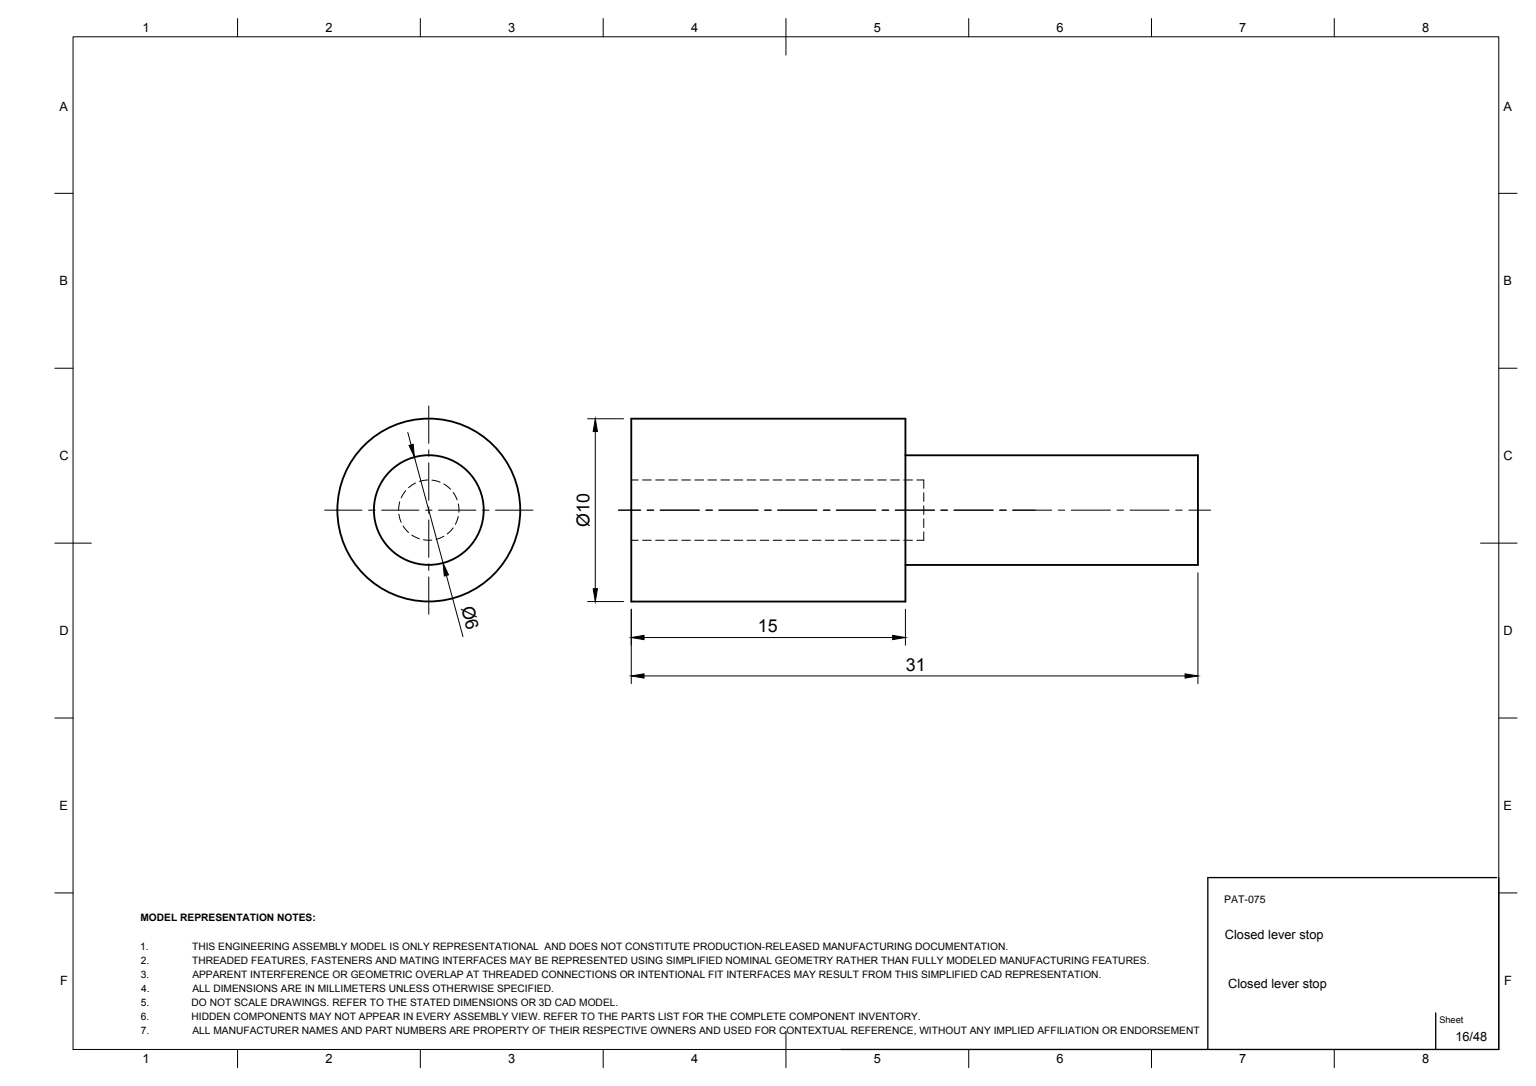
ISO-10303-21;
HEADER;
/* Generated by software containing ST-Developer
 * from STEP Tools, Inc. (www.steptools.com) 
 */

FILE_DESCRIPTION(
/* description */ ('Over-Centre Plunger Toggle Clamp on Slotted Fixture Frame'),
/* implementation_level */ '2;1');

FILE_NAME(
/* name */ 
'Closed lever stop.step',
/* time_stamp */ '2026-10-28T03:23:24-07:00',
/* author */ (''),
/* organization */ (''),
/* preprocessor_version */ 'ST-DEVELOPER v20.2',
/* originating_system */ 'Autodesk Translation Framework v15.17.0.0',
/* authorisation */ '');

FILE_SCHEMA (('AUTOMOTIVE_DESIGN { 1 0 10303 214 3 1 1 }'));
ENDSEC;

DATA;
#10=MECHANICAL_DESIGN_GEOMETRIC_PRESENTATION_REPRESENTATION('',(#524),#15212);
#440=SHAPE_REPRESENTATION_RELATIONSHIP('SRR','None',#15414,#482);
#482=ADVANCED_BREP_SHAPE_REPRESENTATION('',(#575),#15176);
#524=STYLED_ITEM('',(#15712),#575);
#575=MANIFOLD_SOLID_BREP('Body1',#8256);
#712=FACE_BOUND('',#1819,.T.);
#713=FACE_BOUND('',#1822,.T.);
#862=PLANE('',#9048);
#863=PLANE('',#9049);
#864=PLANE('',#9054);
#865=PLANE('',#9057);
#1229=FACE_OUTER_BOUND('',#1816,.T.);
#1230=FACE_OUTER_BOUND('',#1817,.T.);
#1231=FACE_OUTER_BOUND('',#1818,.T.);
#1232=FACE_OUTER_BOUND('',#1820,.T.);
#1233=FACE_OUTER_BOUND('',#1821,.T.);
#1234=FACE_OUTER_BOUND('',#1823,.T.);
#1235=FACE_OUTER_BOUND('',#1824,.T.);
#1816=EDGE_LOOP('',(#6187,#6188,#6189,#6190));
#1817=EDGE_LOOP('',(#6191));
#1818=EDGE_LOOP('',(#6192));
#1819=EDGE_LOOP('',(#6193));
#1820=EDGE_LOOP('',(#6194,#6195,#6196,#6197));
#1821=EDGE_LOOP('',(#6198));
#1822=EDGE_LOOP('',(#6199));
#1823=EDGE_LOOP('',(#6200,#6201,#6202,#6203));
#1824=EDGE_LOOP('',(#6204));
#2414=LINE('',#13041,#3044);
#2415=LINE('',#13052,#3045);
#2416=LINE('',#13056,#3046);
#3044=VECTOR('',#10505,0.165);
#3045=VECTOR('',#10520,0.5);
#3046=VECTOR('',#10525,0.3);
#3617=CIRCLE('',#9046,0.165);
#3618=CIRCLE('',#9047,0.165);
#3619=CIRCLE('',#9050,0.5);
#3620=CIRCLE('',#9051,0.3);
#3621=CIRCLE('',#9053,0.5);
#3622=CIRCLE('',#9056,0.3);
#4065=VERTEX_POINT('',#13038);
#4066=VERTEX_POINT('',#13040);
#4067=VERTEX_POINT('',#13045);
#4068=VERTEX_POINT('',#13047);
#4069=VERTEX_POINT('',#13050);
#4070=VERTEX_POINT('',#13055);
#4854=EDGE_CURVE('',#4065,#4065,#3617,.T.);
#4855=EDGE_CURVE('',#4065,#4066,#2414,.T.);
#4856=EDGE_CURVE('',#4066,#4066,#3618,.T.);
#4857=EDGE_CURVE('',#4067,#4067,#3619,.T.);
#4858=EDGE_CURVE('',#4068,#4068,#3620,.T.);
#4859=EDGE_CURVE('',#4069,#4069,#3621,.T.);
#4860=EDGE_CURVE('',#4069,#4067,#2415,.T.);
#4861=EDGE_CURVE('',#4068,#4070,#2416,.T.);
#4862=EDGE_CURVE('',#4070,#4070,#3622,.T.);
#6187=ORIENTED_EDGE('',*,*,#4854,.F.);
#6188=ORIENTED_EDGE('',*,*,#4855,.T.);
#6189=ORIENTED_EDGE('',*,*,#4856,.F.);
#6190=ORIENTED_EDGE('',*,*,#4855,.F.);
#6191=ORIENTED_EDGE('',*,*,#4854,.T.);
#6192=ORIENTED_EDGE('',*,*,#4857,.F.);
#6193=ORIENTED_EDGE('',*,*,#4858,.T.);
#6194=ORIENTED_EDGE('',*,*,#4859,.F.);
#6195=ORIENTED_EDGE('',*,*,#4860,.T.);
#6196=ORIENTED_EDGE('',*,*,#4857,.T.);
#6197=ORIENTED_EDGE('',*,*,#4860,.F.);
#6198=ORIENTED_EDGE('',*,*,#4859,.T.);
#6199=ORIENTED_EDGE('',*,*,#4856,.T.);
#6200=ORIENTED_EDGE('',*,*,#4858,.F.);
#6201=ORIENTED_EDGE('',*,*,#4861,.T.);
#6202=ORIENTED_EDGE('',*,*,#4862,.T.);
#6203=ORIENTED_EDGE('',*,*,#4861,.F.);
#6204=ORIENTED_EDGE('',*,*,#4862,.F.);
#7680=CYLINDRICAL_SURFACE('',#9045,0.165);
#7681=CYLINDRICAL_SURFACE('',#9052,0.5);
#7682=CYLINDRICAL_SURFACE('',#9055,0.3);
#7901=ADVANCED_FACE('',(#1229),#7680,.F.);
#7902=ADVANCED_FACE('',(#1230),#862,.T.);
#7903=ADVANCED_FACE('',(#1231,#712),#863,.F.);
#7904=ADVANCED_FACE('',(#1232),#7681,.T.);
#7905=ADVANCED_FACE('',(#1233,#713),#864,.T.);
#7906=ADVANCED_FACE('',(#1234),#7682,.T.);
#7907=ADVANCED_FACE('',(#1235),#865,.F.);
#8256=CLOSED_SHELL('',(#7901,#7902,#7903,#7904,#7905,#7906,#7907));
#9044=AXIS2_PLACEMENT_3D('',#13036,#10499,#10500);
#9045=AXIS2_PLACEMENT_3D('',#13037,#10501,#10502);
#9046=AXIS2_PLACEMENT_3D('',#13039,#10503,#10504);
#9047=AXIS2_PLACEMENT_3D('',#13042,#10506,#10507);
#9048=AXIS2_PLACEMENT_3D('',#13043,#10508,#10509);
#9049=AXIS2_PLACEMENT_3D('',#13044,#10510,#10511);
#9050=AXIS2_PLACEMENT_3D('',#13046,#10512,#10513);
#9051=AXIS2_PLACEMENT_3D('',#13048,#10514,#10515);
#9052=AXIS2_PLACEMENT_3D('',#13049,#10516,#10517);
#9053=AXIS2_PLACEMENT_3D('',#13051,#10518,#10519);
#9054=AXIS2_PLACEMENT_3D('',#13053,#10521,#10522);
#9055=AXIS2_PLACEMENT_3D('',#13054,#10523,#10524);
#9056=AXIS2_PLACEMENT_3D('',#13057,#10526,#10527);
#9057=AXIS2_PLACEMENT_3D('',#13058,#10528,#10529);
#10499=DIRECTION('axis',(0.,0.,1.));
#10500=DIRECTION('refdir',(1.,0.,0.));
#10501=DIRECTION('center_axis',(0.,1.,0.));
#10502=DIRECTION('ref_axis',(1.,0.,0.));
#10503=DIRECTION('center_axis',(0.,1.,0.));
#10504=DIRECTION('ref_axis',(1.,0.,0.));
#10505=DIRECTION('',(0.,1.,0.));
#10506=DIRECTION('center_axis',(0.,-1.,0.));
#10507=DIRECTION('ref_axis',(1.,0.,0.));
#10508=DIRECTION('center_axis',(0.,1.,0.));
#10509=DIRECTION('ref_axis',(1.,0.,0.));
#10510=DIRECTION('center_axis',(0.,1.,0.));
#10511=DIRECTION('ref_axis',(1.,0.,0.));
#10512=DIRECTION('center_axis',(0.,1.,0.));
#10513=DIRECTION('ref_axis',(1.,0.,0.));
#10514=DIRECTION('center_axis',(0.,1.,0.));
#10515=DIRECTION('ref_axis',(1.,0.,0.));
#10516=DIRECTION('center_axis',(0.,1.,0.));
#10517=DIRECTION('ref_axis',(1.,0.,0.));
#10518=DIRECTION('center_axis',(0.,1.,0.));
#10519=DIRECTION('ref_axis',(1.,0.,0.));
#10520=DIRECTION('',(0.,-1.,0.));
#10521=DIRECTION('center_axis',(0.,1.,0.));
#10522=DIRECTION('ref_axis',(1.,0.,0.));
#10523=DIRECTION('center_axis',(0.,1.,0.));
#10524=DIRECTION('ref_axis',(1.,0.,0.));
#10525=DIRECTION('',(0.,-1.,0.));
#10526=DIRECTION('center_axis',(0.,1.,0.));
#10527=DIRECTION('ref_axis',(1.,0.,0.));
#10528=DIRECTION('center_axis',(0.,1.,0.));
#10529=DIRECTION('ref_axis',(1.,0.,0.));
#13036=CARTESIAN_POINT('',(0.,0.,0.));
#13037=CARTESIAN_POINT('Origin',(-5.25982293614231,-2.4,14.8604204653858));
#13038=CARTESIAN_POINT('',(-5.42482293614231,-2.4,14.8604204653858));
#13039=CARTESIAN_POINT('Origin',(-5.25982293614231,-2.4,14.8604204653858));
#13040=CARTESIAN_POINT('',(-5.42482293614231,-0.8,14.8604204653858));
#13041=CARTESIAN_POINT('',(-5.42482293614231,-2.4,14.8604204653858));
#13042=CARTESIAN_POINT('Origin',(-5.25982293614231,-0.8,14.8604204653858));
#13043=CARTESIAN_POINT('Origin',(-5.25982293614231,-2.4,14.8604204653858));
#13044=CARTESIAN_POINT('Origin',(-5.25982293614231,-2.3,14.8604204653858));
#13045=CARTESIAN_POINT('',(-5.75982293614231,-2.3,14.8604204653858));
#13046=CARTESIAN_POINT('Origin',(-5.25982293614231,-2.3,14.8604204653858));
#13047=CARTESIAN_POINT('',(-5.55982293614231,-2.3,14.8604204653858));
#13048=CARTESIAN_POINT('Origin',(-5.25982293614231,-2.3,14.8604204653858));
#13049=CARTESIAN_POINT('Origin',(-5.25982293614231,-2.3,14.8604204653858));
#13050=CARTESIAN_POINT('',(-5.75982293614231,-0.8,14.8604204653858));
#13051=CARTESIAN_POINT('Origin',(-5.25982293614231,-0.8,14.8604204653858));
#13052=CARTESIAN_POINT('',(-5.75982293614231,-2.3,14.8604204653858));
#13053=CARTESIAN_POINT('Origin',(-5.25982293614231,-0.8,14.8604204653858));
#13054=CARTESIAN_POINT('Origin',(-5.25982293614231,-3.9,14.8604204653858));
#13055=CARTESIAN_POINT('',(-5.55982293614231,-3.9,14.8604204653858));
#13056=CARTESIAN_POINT('',(-5.55982293614231,-3.9,14.8604204653858));
#13057=CARTESIAN_POINT('Origin',(-5.25982293614231,-3.9,14.8604204653858));
#13058=CARTESIAN_POINT('Origin',(-5.25982293614231,-3.9,14.8604204653858));
#15126=UNCERTAINTY_MEASURE_WITH_UNIT(LENGTH_MEASURE(0.001),#15213,
'DISTANCE_ACCURACY_VALUE',
'Maximum model space distance between geometric entities at asserted c
onnectivities');
#15162=UNCERTAINTY_MEASURE_WITH_UNIT(LENGTH_MEASURE(0.001),#15213,
'DISTANCE_ACCURACY_VALUE',
'Maximum model space distance between geometric entities at asserted c
onnectivities');
#15176=(
GEOMETRIC_REPRESENTATION_CONTEXT(3)
GLOBAL_UNCERTAINTY_ASSIGNED_CONTEXT((#15126))
GLOBAL_UNIT_ASSIGNED_CONTEXT((#15213,#15215,#15216))
REPRESENTATION_CONTEXT('','3D')
);
#15212=(
GEOMETRIC_REPRESENTATION_CONTEXT(3)
GLOBAL_UNCERTAINTY_ASSIGNED_CONTEXT((#15162))
GLOBAL_UNIT_ASSIGNED_CONTEXT((#15213,#15215,#15216))
REPRESENTATION_CONTEXT('','3D')
);
#15213=(
LENGTH_UNIT()
NAMED_UNIT(*)
SI_UNIT(.CENTI.,.METRE.)
);
#15215=(
NAMED_UNIT(*)
PLANE_ANGLE_UNIT()
SI_UNIT($,.RADIAN.)
);
#15216=(
NAMED_UNIT(*)
SI_UNIT($,.STERADIAN.)
SOLID_ANGLE_UNIT()
);
#15230=SHAPE_DEFINITION_REPRESENTATION(#15279,#15414);
#15279=PRODUCT_DEFINITION_SHAPE('',$,#15464);
#15414=SHAPE_REPRESENTATION('',(#9044),#15176);
#15450=PRODUCT_DEFINITION_CONTEXT('part definition',#15599,'design');
#15464=PRODUCT_DEFINITION('Closed lever stop','Closed lever stop',#15513,
#15450);
#15513=PRODUCT_DEFINITION_FORMATION('',$,#15614);
#15599=APPLICATION_CONTEXT(
'Core Data for Automotive Mechanical Design Process');
#15600=PRODUCT_CONTEXT('part definition',#15599,'mechanical');
#15614=PRODUCT('Closed lever stop','Closed lever stop',
'Closed lever stop',(#15600));
#15706=COLOUR_RGB('Sky Blue',0.24,0.69,0.87);
#15707=FILL_AREA_STYLE_COLOUR('',#15706);
#15708=FILL_AREA_STYLE('',(#15707));
#15709=SURFACE_STYLE_FILL_AREA(#15708);
#15710=SURFACE_SIDE_STYLE('',(#15709));
#15711=SURFACE_STYLE_USAGE(.BOTH.,#15710);
#15712=PRESENTATION_STYLE_ASSIGNMENT((#15711));
ENDSEC;
END-ISO-10303-21;
